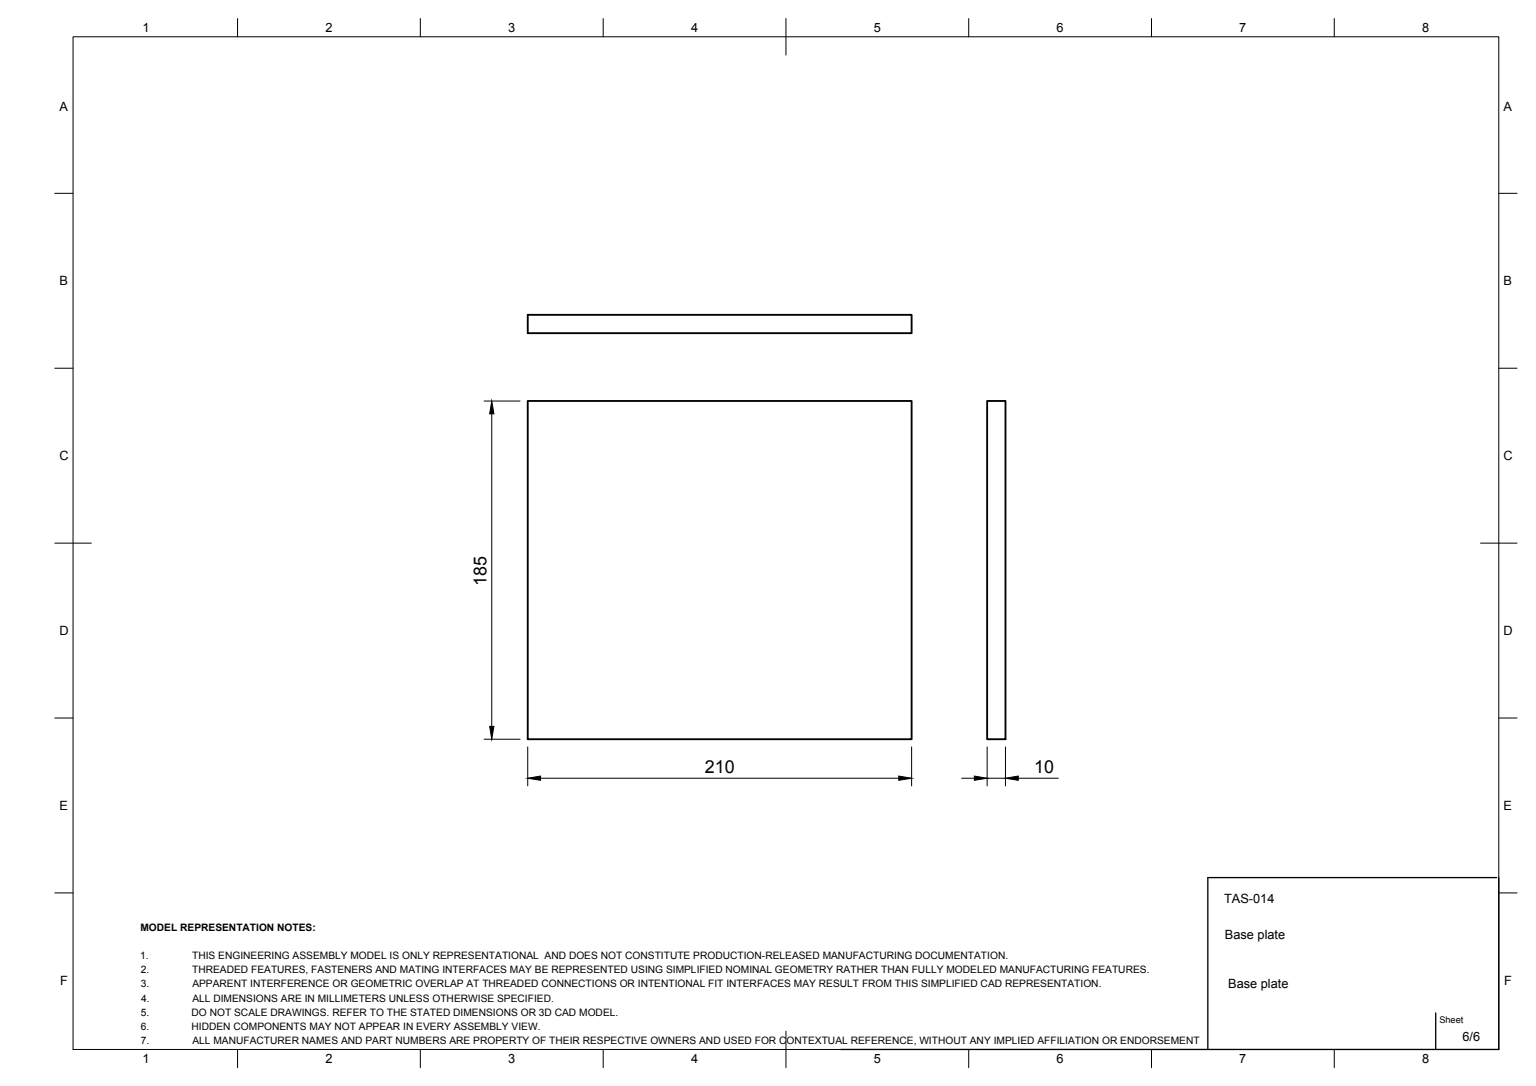
ISO-10303-21;
HEADER;
/* Generated by software containing ST-Developer
 * from STEP Tools, Inc. (www.steptools.com) 
 */

FILE_DESCRIPTION(
/* description */ ('STEP AP214'),
/* implementation_level */ '2;1');

FILE_NAME(
/* name */ 'Base Plate.step',
/* time_stamp */ '2026-11-15T15:22:30-08:00',
/* author */ (''),
/* organization */ (''),
/* preprocessor_version */ 'ST-DEVELOPER v20.2',
/* originating_system */ 'Autodesk Translation Framework v15.17.0.0',
/* authorisation */ '');

FILE_SCHEMA (('AUTOMOTIVE_DESIGN { 1 0 10303 214 3 1 1 }'));
ENDSEC;

DATA;
#10=MECHANICAL_DESIGN_GEOMETRIC_PRESENTATION_REPRESENTATION('',(#86),#3119);
#69=SHAPE_REPRESENTATION_RELATIONSHIP('SRR','None',#3151,#73);
#73=ADVANCED_BREP_SHAPE_REPRESENTATION('',(#93),#3117);
#86=STYLED_ITEM('',(#3178),#93);
#93=MANIFOLD_SOLID_BREP('Body1',#1805);
#287=FACE_OUTER_BOUND('',#388,.T.);
#288=FACE_OUTER_BOUND('',#389,.T.);
#289=FACE_OUTER_BOUND('',#390,.T.);
#290=FACE_OUTER_BOUND('',#391,.T.);
#291=FACE_OUTER_BOUND('',#392,.T.);
#292=FACE_OUTER_BOUND('',#393,.T.);
#388=EDGE_LOOP('',(#1592,#1593,#1594,#1595));
#389=EDGE_LOOP('',(#1596,#1597,#1598,#1599));
#390=EDGE_LOOP('',(#1600,#1601,#1602,#1603));
#391=EDGE_LOOP('',(#1604,#1605,#1606,#1607));
#392=EDGE_LOOP('',(#1608,#1609,#1610,#1611));
#393=EDGE_LOOP('',(#1612,#1613,#1614,#1615));
#549=LINE('',#3038,#724);
#550=LINE('',#3040,#725);
#551=LINE('',#3042,#726);
#552=LINE('',#3043,#727);
#553=LINE('',#3046,#728);
#554=LINE('',#3048,#729);
#555=LINE('',#3049,#730);
#556=LINE('',#3052,#731);
#557=LINE('',#3054,#732);
#558=LINE('',#3055,#733);
#559=LINE('',#3057,#734);
#560=LINE('',#3058,#735);
#724=VECTOR('',#2498,1000.);
#725=VECTOR('',#2499,1000.);
#726=VECTOR('',#2500,1000.);
#727=VECTOR('',#2501,1000.);
#728=VECTOR('',#2504,1000.);
#729=VECTOR('',#2505,1000.);
#730=VECTOR('',#2506,1000.);
#731=VECTOR('',#2509,1000.);
#732=VECTOR('',#2510,1000.);
#733=VECTOR('',#2511,1000.);
#734=VECTOR('',#2514,1000.);
#735=VECTOR('',#2515,1000.);
#903=VERTEX_POINT('',#3036);
#904=VERTEX_POINT('',#3037);
#905=VERTEX_POINT('',#3039);
#906=VERTEX_POINT('',#3041);
#907=VERTEX_POINT('',#3045);
#908=VERTEX_POINT('',#3047);
#909=VERTEX_POINT('',#3051);
#910=VERTEX_POINT('',#3053);
#1141=EDGE_CURVE('',#903,#904,#549,.T.);
#1142=EDGE_CURVE('',#905,#904,#550,.T.);
#1143=EDGE_CURVE('',#906,#905,#551,.T.);
#1144=EDGE_CURVE('',#906,#903,#552,.T.);
#1145=EDGE_CURVE('',#904,#907,#553,.T.);
#1146=EDGE_CURVE('',#908,#907,#554,.T.);
#1147=EDGE_CURVE('',#905,#908,#555,.T.);
#1148=EDGE_CURVE('',#907,#909,#556,.T.);
#1149=EDGE_CURVE('',#910,#909,#557,.T.);
#1150=EDGE_CURVE('',#908,#910,#558,.T.);
#1151=EDGE_CURVE('',#909,#903,#559,.T.);
#1152=EDGE_CURVE('',#910,#906,#560,.T.);
#1592=ORIENTED_EDGE('',*,*,#1141,.T.);
#1593=ORIENTED_EDGE('',*,*,#1142,.F.);
#1594=ORIENTED_EDGE('',*,*,#1143,.F.);
#1595=ORIENTED_EDGE('',*,*,#1144,.T.);
#1596=ORIENTED_EDGE('',*,*,#1145,.T.);
#1597=ORIENTED_EDGE('',*,*,#1146,.F.);
#1598=ORIENTED_EDGE('',*,*,#1147,.F.);
#1599=ORIENTED_EDGE('',*,*,#1142,.T.);
#1600=ORIENTED_EDGE('',*,*,#1148,.T.);
#1601=ORIENTED_EDGE('',*,*,#1149,.F.);
#1602=ORIENTED_EDGE('',*,*,#1150,.F.);
#1603=ORIENTED_EDGE('',*,*,#1146,.T.);
#1604=ORIENTED_EDGE('',*,*,#1151,.T.);
#1605=ORIENTED_EDGE('',*,*,#1144,.F.);
#1606=ORIENTED_EDGE('',*,*,#1152,.F.);
#1607=ORIENTED_EDGE('',*,*,#1149,.T.);
#1608=ORIENTED_EDGE('',*,*,#1143,.T.);
#1609=ORIENTED_EDGE('',*,*,#1147,.T.);
#1610=ORIENTED_EDGE('',*,*,#1150,.T.);
#1611=ORIENTED_EDGE('',*,*,#1152,.T.);
#1612=ORIENTED_EDGE('',*,*,#1141,.F.);
#1613=ORIENTED_EDGE('',*,*,#1151,.F.);
#1614=ORIENTED_EDGE('',*,*,#1148,.F.);
#1615=ORIENTED_EDGE('',*,*,#1145,.F.);
#1694=PLANE('',#2008);
#1695=PLANE('',#2009);
#1696=PLANE('',#2010);
#1697=PLANE('',#2011);
#1698=PLANE('',#2012);
#1699=PLANE('',#2013);
#1787=ADVANCED_FACE('',(#287),#1694,.F.);
#1788=ADVANCED_FACE('',(#288),#1695,.F.);
#1789=ADVANCED_FACE('',(#289),#1696,.F.);
#1790=ADVANCED_FACE('',(#290),#1697,.F.);
#1791=ADVANCED_FACE('',(#291),#1698,.F.);
#1792=ADVANCED_FACE('',(#292),#1699,.T.);
#1805=CLOSED_SHELL('',(#1787,#1788,#1789,#1790,#1791,#1792));
#2007=AXIS2_PLACEMENT_3D('',#3034,#2494,#2495);
#2008=AXIS2_PLACEMENT_3D('',#3035,#2496,#2497);
#2009=AXIS2_PLACEMENT_3D('',#3044,#2502,#2503);
#2010=AXIS2_PLACEMENT_3D('',#3050,#2507,#2508);
#2011=AXIS2_PLACEMENT_3D('',#3056,#2512,#2513);
#2012=AXIS2_PLACEMENT_3D('',#3059,#2516,#2517);
#2013=AXIS2_PLACEMENT_3D('',#3060,#2518,#2519);
#2494=DIRECTION('axis',(0.,0.,1.));
#2495=DIRECTION('refdir',(1.,0.,0.));
#2496=DIRECTION('center_axis',(-1.,0.,0.));
#2497=DIRECTION('ref_axis',(0.,0.,1.));
#2498=DIRECTION('',(0.,1.,0.));
#2499=DIRECTION('',(0.,0.,-1.));
#2500=DIRECTION('',(0.,1.,0.));
#2501=DIRECTION('',(0.,0.,-1.));
#2502=DIRECTION('center_axis',(0.,-1.,0.));
#2503=DIRECTION('ref_axis',(0.,0.,-1.));
#2504=DIRECTION('',(-1.,0.,0.));
#2505=DIRECTION('',(0.,0.,-1.));
#2506=DIRECTION('',(-1.,0.,0.));
#2507=DIRECTION('center_axis',(1.,0.,0.));
#2508=DIRECTION('ref_axis',(0.,0.,-1.));
#2509=DIRECTION('',(0.,-1.,0.));
#2510=DIRECTION('',(0.,0.,-1.));
#2511=DIRECTION('',(0.,-1.,0.));
#2512=DIRECTION('center_axis',(0.,1.,0.));
#2513=DIRECTION('ref_axis',(0.,0.,1.));
#2514=DIRECTION('',(1.,0.,0.));
#2515=DIRECTION('',(1.,0.,0.));
#2516=DIRECTION('center_axis',(0.,0.,-1.));
#2517=DIRECTION('ref_axis',(-1.,0.,0.));
#2518=DIRECTION('center_axis',(0.,0.,-1.));
#2519=DIRECTION('ref_axis',(-1.,0.,0.));
#3034=CARTESIAN_POINT('',(0.,0.,0.));
#3035=CARTESIAN_POINT('Origin',(105.,-92.5,5.));
#3036=CARTESIAN_POINT('',(105.,-92.5,-5.));
#3037=CARTESIAN_POINT('',(105.,92.5,-5.));
#3038=CARTESIAN_POINT('',(105.,-92.5,-5.));
#3039=CARTESIAN_POINT('',(105.,92.5,5.));
#3040=CARTESIAN_POINT('',(105.,92.5,5.));
#3041=CARTESIAN_POINT('',(105.,-92.5,5.));
#3042=CARTESIAN_POINT('',(105.,-92.5,5.));
#3043=CARTESIAN_POINT('',(105.,-92.5,5.));
#3044=CARTESIAN_POINT('Origin',(-105.,92.5,5.));
#3045=CARTESIAN_POINT('',(-105.,92.5,-5.));
#3046=CARTESIAN_POINT('',(-105.,92.5,-5.));
#3047=CARTESIAN_POINT('',(-105.,92.5,5.));
#3048=CARTESIAN_POINT('',(-105.,92.5,5.));
#3049=CARTESIAN_POINT('',(-105.,92.5,5.));
#3050=CARTESIAN_POINT('Origin',(-105.,-92.5,5.));
#3051=CARTESIAN_POINT('',(-105.,-92.5,-5.));
#3052=CARTESIAN_POINT('',(-105.,-92.5,-5.));
#3053=CARTESIAN_POINT('',(-105.,-92.5,5.));
#3054=CARTESIAN_POINT('',(-105.,-92.5,5.));
#3055=CARTESIAN_POINT('',(-105.,-92.5,5.));
#3056=CARTESIAN_POINT('Origin',(-105.,-92.5,5.));
#3057=CARTESIAN_POINT('',(-105.,-92.5,-5.));
#3058=CARTESIAN_POINT('',(-105.,-92.5,5.));
#3059=CARTESIAN_POINT('Origin',(0.,0.,5.));
#3060=CARTESIAN_POINT('Origin',(0.,0.,-5.));
#3111=UNCERTAINTY_MEASURE_WITH_UNIT(LENGTH_MEASURE(0.01),#3120,
'DISTANCE_ACCURACY_VALUE',
'Maximum model space distance between geometric entities at asserted c
onnectivities');
#3113=UNCERTAINTY_MEASURE_WITH_UNIT(LENGTH_MEASURE(0.01),#3120,
'DISTANCE_ACCURACY_VALUE',
'Maximum model space distance between geometric entities at asserted c
onnectivities');
#3117=(
GEOMETRIC_REPRESENTATION_CONTEXT(3)
GLOBAL_UNCERTAINTY_ASSIGNED_CONTEXT((#3111))
GLOBAL_UNIT_ASSIGNED_CONTEXT((#3120,#3122,#3123))
REPRESENTATION_CONTEXT('','3D')
);
#3119=(
GEOMETRIC_REPRESENTATION_CONTEXT(3)
GLOBAL_UNCERTAINTY_ASSIGNED_CONTEXT((#3113))
GLOBAL_UNIT_ASSIGNED_CONTEXT((#3120,#3122,#3123))
REPRESENTATION_CONTEXT('','3D')
);
#3120=(
LENGTH_UNIT()
NAMED_UNIT(*)
SI_UNIT(.MILLI.,.METRE.)
);
#3122=(
NAMED_UNIT(*)
PLANE_ANGLE_UNIT()
SI_UNIT($,.RADIAN.)
);
#3123=(
NAMED_UNIT(*)
SI_UNIT($,.STERADIAN.)
SOLID_ANGLE_UNIT()
);
#3127=SHAPE_DEFINITION_REPRESENTATION(#3132,#3151);
#3132=PRODUCT_DEFINITION_SHAPE('',$,#3157);
#3151=SHAPE_REPRESENTATION('',(#2007),#3117);
#3153=PRODUCT_DEFINITION_CONTEXT('part definition',#3170,'design');
#3157=PRODUCT_DEFINITION('Base plate','Base Plate',#3162,#3153);
#3162=PRODUCT_DEFINITION_FORMATION('',$,#3175);
#3170=APPLICATION_CONTEXT(
'Core Data for Automotive Mechanical Design Process');
#3171=PRODUCT_CONTEXT('part definition',#3170,'mechanical');
#3175=PRODUCT('Base plate','Base Plate','Base plate',(#3171));
#3178=PRESENTATION_STYLE_ASSIGNMENT((#3180));
#3180=SURFACE_STYLE_USAGE(.BOTH.,#3182);
#3182=SURFACE_SIDE_STYLE('',(#3184));
#3184=SURFACE_STYLE_FILL_AREA(#3186);
#3186=FILL_AREA_STYLE('Opaque(202,209,238)',(#3188));
#3188=FILL_AREA_STYLE_COLOUR('Opaque(202,209,238)',#3190);
#3190=COLOUR_RGB('Opaque(202,209,238)',0.792156862745098,0.819607843137255,
0.933333333333333);
ENDSEC;
END-ISO-10303-21;
